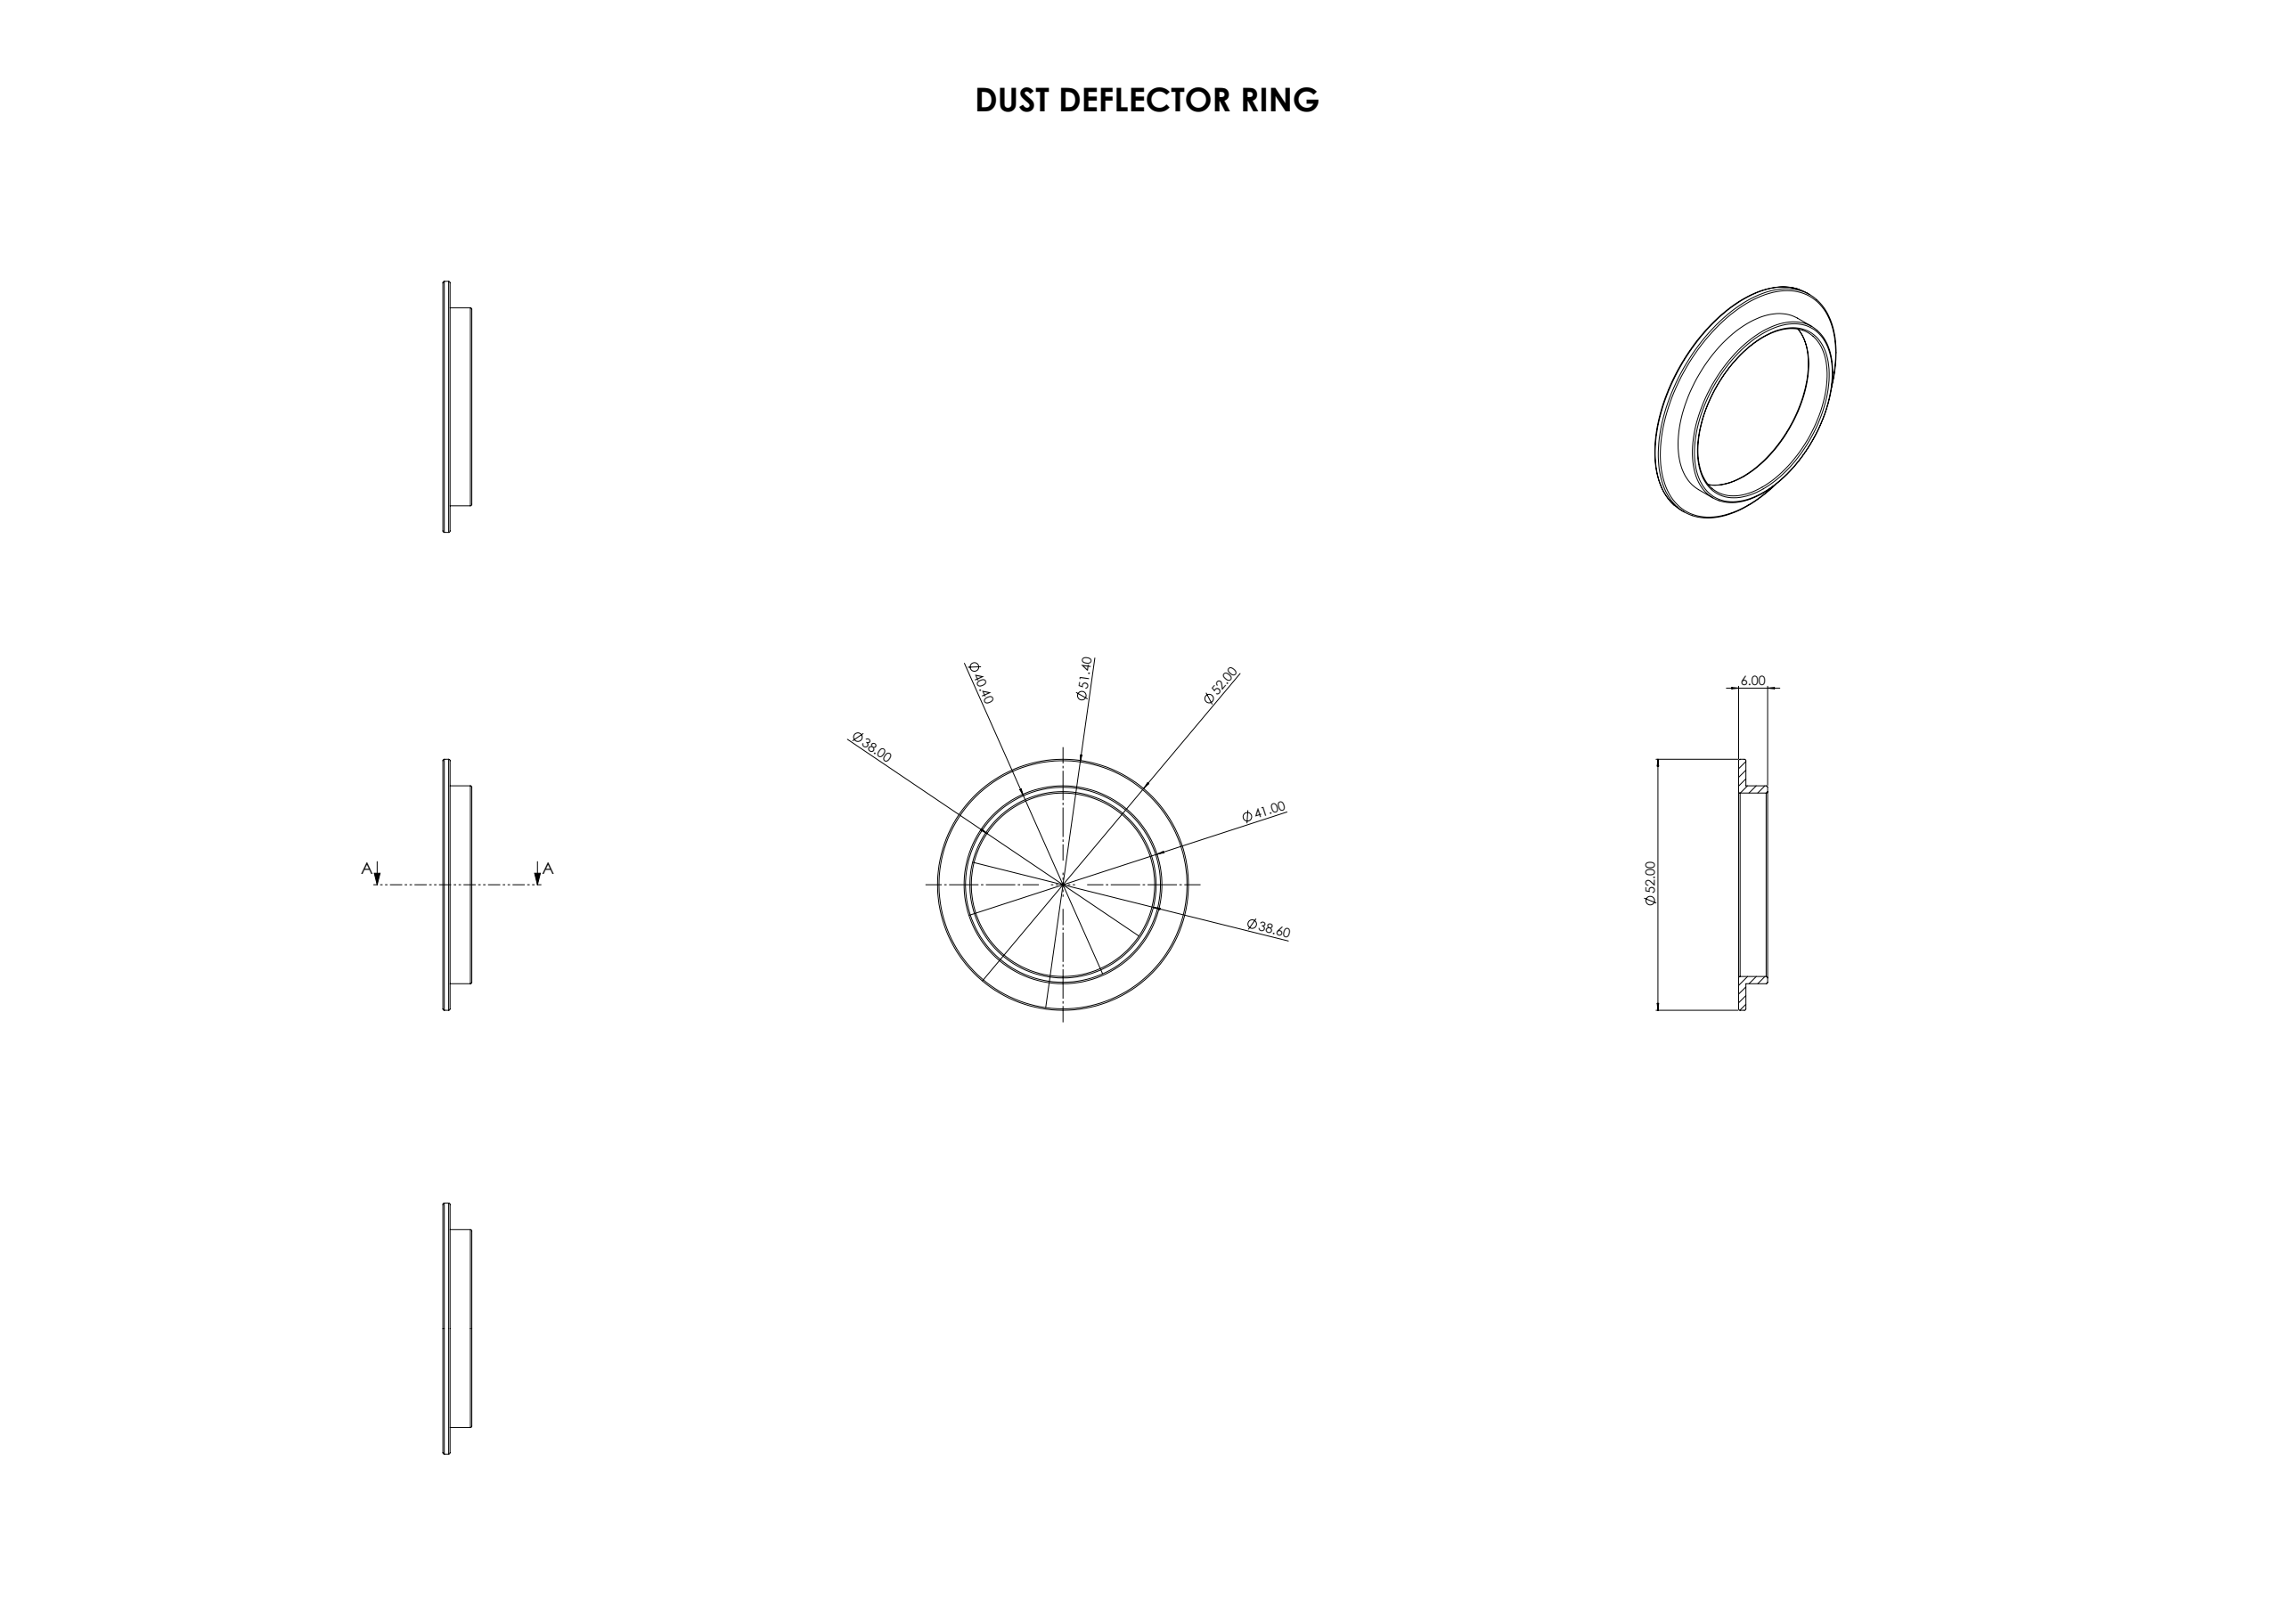
ISO-10303-21;
HEADER;
/* Generated by software containing ST-Developer
 * from STEP Tools, Inc. (www.steptools.com) 
 */

FILE_DESCRIPTION(
/* description */ (''),
/* implementation_level */ '2;1');

FILE_NAME(
/* name */ '16_Dust_Deflector_Ring.step',
/* time_stamp */ '2026-10-11T12:57:03-07:00',
/* author */ (''),
/* organization */ (''),
/* preprocessor_version */ 'ST-DEVELOPER v20.2',
/* originating_system */ 'Autodesk Translation Framework v15.15.0.0',
/* authorisation */ '');

FILE_SCHEMA (('AUTOMOTIVE_DESIGN { 1 0 10303 214 3 1 1 }'));
ENDSEC;

DATA;
#10=MECHANICAL_DESIGN_GEOMETRIC_PRESENTATION_REPRESENTATION('',(#271),#90374);
#237=SHAPE_REPRESENTATION_RELATIONSHIP('SRR','None',#90456,#254);
#254=ADVANCED_BREP_SHAPE_REPRESENTATION('',(#288),#90372);
#271=STYLED_ITEM('',(#90673),#288);
#288=MANIFOLD_SOLID_BREP('Body1',#40360);
#1035=TOROIDAL_SURFACE('',#45228,19.3,0.3);
#1036=TOROIDAL_SURFACE('',#45238,19.3,0.3);
#1037=TOROIDAL_SURFACE('',#45243,20.2,0.3);
#1038=TOROIDAL_SURFACE('',#45249,25.7,0.3);
#1039=TOROIDAL_SURFACE('',#45258,25.7,0.3);
#1113=FACE_BOUND('',#6998,.T.);
#1114=FACE_BOUND('',#7001,.T.);
#1115=FACE_BOUND('',#7007,.T.);
#1821=PLANE('',#45236);
#1822=PLANE('',#45241);
#1823=PLANE('',#45257);
#4525=FACE_OUTER_BOUND('',#6995,.T.);
#4526=FACE_OUTER_BOUND('',#6996,.T.);
#4527=FACE_OUTER_BOUND('',#6997,.T.);
#4528=FACE_OUTER_BOUND('',#6999,.T.);
#4529=FACE_OUTER_BOUND('',#7000,.T.);
#4530=FACE_OUTER_BOUND('',#7002,.T.);
#4531=FACE_OUTER_BOUND('',#7003,.T.);
#4532=FACE_OUTER_BOUND('',#7004,.T.);
#4533=FACE_OUTER_BOUND('',#7005,.T.);
#4534=FACE_OUTER_BOUND('',#7006,.T.);
#4535=FACE_OUTER_BOUND('',#7008,.T.);
#6995=EDGE_LOOP('',(#37155,#37156,#37157,#37158,#37159));
#6996=EDGE_LOOP('',(#37160,#37161,#37162,#37163,#37164,#37165));
#6997=EDGE_LOOP('',(#37166));
#6998=EDGE_LOOP('',(#37167));
#6999=EDGE_LOOP('',(#37168,#37169,#37170,#37171,#37172));
#7000=EDGE_LOOP('',(#37173));
#7001=EDGE_LOOP('',(#37174));
#7002=EDGE_LOOP('',(#37175,#37176,#37177,#37178,#37179));
#7003=EDGE_LOOP('',(#37180,#37181,#37182,#37183,#37184));
#7004=EDGE_LOOP('',(#37185,#37186,#37187,#37188,#37189));
#7005=EDGE_LOOP('',(#37190,#37191,#37192,#37193,#37194,#37195));
#7006=EDGE_LOOP('',(#37196));
#7007=EDGE_LOOP('',(#37197));
#7008=EDGE_LOOP('',(#37198,#37199,#37200,#37201,#37202));
#9399=CIRCLE('',#45229,19.3);
#9400=CIRCLE('',#45230,0.3);
#9401=CIRCLE('',#45231,19.);
#9402=CIRCLE('',#45232,19.);
#9403=CIRCLE('',#45234,19.);
#9404=CIRCLE('',#45235,19.);
#9405=CIRCLE('',#45237,25.7);
#9406=CIRCLE('',#45239,0.3);
#9407=CIRCLE('',#45240,19.3);
#9408=CIRCLE('',#45242,20.2);
#9409=CIRCLE('',#45244,0.3);
#9410=CIRCLE('',#45245,20.5);
#9411=CIRCLE('',#45246,20.5);
#9412=CIRCLE('',#45248,20.5);
#9413=CIRCLE('',#45250,25.7);
#9414=CIRCLE('',#45251,0.3);
#9415=CIRCLE('',#45252,26.);
#9416=CIRCLE('',#45253,26.);
#9417=CIRCLE('',#45255,26.);
#9418=CIRCLE('',#45256,26.);
#9419=CIRCLE('',#45259,0.3);
#12841=LINE('',#90247,#15335);
#12842=LINE('',#90266,#15336);
#12843=LINE('',#90278,#15337);
#15335=VECTOR('',#57151,19.);
#15336=VECTOR('',#57176,20.5);
#15337=VECTOR('',#57191,26.);
#19050=VERTEX_POINT('',#90235);
#19051=VERTEX_POINT('',#90237);
#19052=VERTEX_POINT('',#90239);
#19053=VERTEX_POINT('',#90243);
#19054=VERTEX_POINT('',#90244);
#19055=VERTEX_POINT('',#90249);
#19056=VERTEX_POINT('',#90252);
#19057=VERTEX_POINT('',#90256);
#19058=VERTEX_POINT('',#90259);
#19059=VERTEX_POINT('',#90261);
#19060=VERTEX_POINT('',#90265);
#19061=VERTEX_POINT('',#90269);
#19062=VERTEX_POINT('',#90271);
#19063=VERTEX_POINT('',#90273);
#19064=VERTEX_POINT('',#90277);
#19065=VERTEX_POINT('',#90279);
#25089=EDGE_CURVE('',#19050,#19050,#9399,.T.);
#25090=EDGE_CURVE('',#19050,#19051,#9400,.T.);
#25091=EDGE_CURVE('',#19051,#19052,#9401,.T.);
#25092=EDGE_CURVE('',#19052,#19051,#9402,.T.);
#25093=EDGE_CURVE('',#19053,#19054,#9403,.T.);
#25094=EDGE_CURVE('',#19054,#19053,#9404,.T.);
#25095=EDGE_CURVE('',#19054,#19052,#12841,.T.);
#25096=EDGE_CURVE('',#19055,#19055,#9405,.T.);
#25097=EDGE_CURVE('',#19053,#19056,#9406,.T.);
#25098=EDGE_CURVE('',#19056,#19056,#9407,.T.);
#25099=EDGE_CURVE('',#19057,#19057,#9408,.T.);
#25100=EDGE_CURVE('',#19057,#19058,#9409,.T.);
#25101=EDGE_CURVE('',#19058,#19059,#9410,.T.);
#25102=EDGE_CURVE('',#19059,#19058,#9411,.T.);
#25103=EDGE_CURVE('',#19059,#19060,#12842,.T.);
#25104=EDGE_CURVE('',#19060,#19060,#9412,.T.);
#25105=EDGE_CURVE('',#19061,#19061,#9413,.T.);
#25106=EDGE_CURVE('',#19061,#19062,#9414,.T.);
#25107=EDGE_CURVE('',#19062,#19063,#9415,.T.);
#25108=EDGE_CURVE('',#19063,#19062,#9416,.T.);
#25109=EDGE_CURVE('',#19063,#19064,#12843,.T.);
#25110=EDGE_CURVE('',#19065,#19064,#9417,.T.);
#25111=EDGE_CURVE('',#19064,#19065,#9418,.T.);
#25112=EDGE_CURVE('',#19065,#19055,#9419,.T.);
#37155=ORIENTED_EDGE('',*,*,#25089,.T.);
#37156=ORIENTED_EDGE('',*,*,#25090,.T.);
#37157=ORIENTED_EDGE('',*,*,#25091,.T.);
#37158=ORIENTED_EDGE('',*,*,#25092,.T.);
#37159=ORIENTED_EDGE('',*,*,#25090,.F.);
#37160=ORIENTED_EDGE('',*,*,#25093,.F.);
#37161=ORIENTED_EDGE('',*,*,#25094,.F.);
#37162=ORIENTED_EDGE('',*,*,#25095,.T.);
#37163=ORIENTED_EDGE('',*,*,#25091,.F.);
#37164=ORIENTED_EDGE('',*,*,#25092,.F.);
#37165=ORIENTED_EDGE('',*,*,#25095,.F.);
#37166=ORIENTED_EDGE('',*,*,#25096,.F.);
#37167=ORIENTED_EDGE('',*,*,#25089,.F.);
#37168=ORIENTED_EDGE('',*,*,#25093,.T.);
#37169=ORIENTED_EDGE('',*,*,#25094,.T.);
#37170=ORIENTED_EDGE('',*,*,#25097,.T.);
#37171=ORIENTED_EDGE('',*,*,#25098,.T.);
#37172=ORIENTED_EDGE('',*,*,#25097,.F.);
#37173=ORIENTED_EDGE('',*,*,#25099,.F.);
#37174=ORIENTED_EDGE('',*,*,#25098,.F.);
#37175=ORIENTED_EDGE('',*,*,#25099,.T.);
#37176=ORIENTED_EDGE('',*,*,#25100,.T.);
#37177=ORIENTED_EDGE('',*,*,#25101,.T.);
#37178=ORIENTED_EDGE('',*,*,#25102,.T.);
#37179=ORIENTED_EDGE('',*,*,#25100,.F.);
#37180=ORIENTED_EDGE('',*,*,#25102,.F.);
#37181=ORIENTED_EDGE('',*,*,#25103,.T.);
#37182=ORIENTED_EDGE('',*,*,#25104,.T.);
#37183=ORIENTED_EDGE('',*,*,#25103,.F.);
#37184=ORIENTED_EDGE('',*,*,#25101,.F.);
#37185=ORIENTED_EDGE('',*,*,#25105,.T.);
#37186=ORIENTED_EDGE('',*,*,#25106,.T.);
#37187=ORIENTED_EDGE('',*,*,#25107,.T.);
#37188=ORIENTED_EDGE('',*,*,#25108,.T.);
#37189=ORIENTED_EDGE('',*,*,#25106,.F.);
#37190=ORIENTED_EDGE('',*,*,#25108,.F.);
#37191=ORIENTED_EDGE('',*,*,#25109,.T.);
#37192=ORIENTED_EDGE('',*,*,#25110,.F.);
#37193=ORIENTED_EDGE('',*,*,#25111,.F.);
#37194=ORIENTED_EDGE('',*,*,#25109,.F.);
#37195=ORIENTED_EDGE('',*,*,#25107,.F.);
#37196=ORIENTED_EDGE('',*,*,#25105,.F.);
#37197=ORIENTED_EDGE('',*,*,#25104,.F.);
#37198=ORIENTED_EDGE('',*,*,#25110,.T.);
#37199=ORIENTED_EDGE('',*,*,#25111,.T.);
#37200=ORIENTED_EDGE('',*,*,#25112,.T.);
#37201=ORIENTED_EDGE('',*,*,#25096,.T.);
#37202=ORIENTED_EDGE('',*,*,#25112,.F.);
#37943=CYLINDRICAL_SURFACE('',#45233,19.);
#37944=CYLINDRICAL_SURFACE('',#45247,20.5);
#37945=CYLINDRICAL_SURFACE('',#45254,26.);
#40328=ADVANCED_FACE('',(#4525),#1035,.T.);
#40329=ADVANCED_FACE('',(#4526),#37943,.F.);
#40330=ADVANCED_FACE('',(#4527,#1113),#1821,.T.);
#40331=ADVANCED_FACE('',(#4528),#1036,.T.);
#40332=ADVANCED_FACE('',(#4529,#1114),#1822,.T.);
#40333=ADVANCED_FACE('',(#4530),#1037,.T.);
#40334=ADVANCED_FACE('',(#4531),#37944,.T.);
#40335=ADVANCED_FACE('',(#4532),#1038,.T.);
#40336=ADVANCED_FACE('',(#4533),#37945,.T.);
#40337=ADVANCED_FACE('',(#4534,#1115),#1823,.T.);
#40338=ADVANCED_FACE('',(#4535),#1039,.T.);
#40360=CLOSED_SHELL('',(#40328,#40329,#40330,#40331,#40332,#40333,#40334,
#40335,#40336,#40337,#40338));
#45227=AXIS2_PLACEMENT_3D('',#90233,#57133,#57134);
#45228=AXIS2_PLACEMENT_3D('',#90234,#57135,#57136);
#45229=AXIS2_PLACEMENT_3D('',#90236,#57137,#57138);
#45230=AXIS2_PLACEMENT_3D('',#90238,#57139,#57140);
#45231=AXIS2_PLACEMENT_3D('',#90240,#57141,#57142);
#45232=AXIS2_PLACEMENT_3D('',#90241,#57143,#57144);
#45233=AXIS2_PLACEMENT_3D('',#90242,#57145,#57146);
#45234=AXIS2_PLACEMENT_3D('',#90245,#57147,#57148);
#45235=AXIS2_PLACEMENT_3D('',#90246,#57149,#57150);
#45236=AXIS2_PLACEMENT_3D('',#90248,#57152,#57153);
#45237=AXIS2_PLACEMENT_3D('',#90250,#57154,#57155);
#45238=AXIS2_PLACEMENT_3D('',#90251,#57156,#57157);
#45239=AXIS2_PLACEMENT_3D('',#90253,#57158,#57159);
#45240=AXIS2_PLACEMENT_3D('',#90254,#57160,#57161);
#45241=AXIS2_PLACEMENT_3D('',#90255,#57162,#57163);
#45242=AXIS2_PLACEMENT_3D('',#90257,#57164,#57165);
#45243=AXIS2_PLACEMENT_3D('',#90258,#57166,#57167);
#45244=AXIS2_PLACEMENT_3D('',#90260,#57168,#57169);
#45245=AXIS2_PLACEMENT_3D('',#90262,#57170,#57171);
#45246=AXIS2_PLACEMENT_3D('',#90263,#57172,#57173);
#45247=AXIS2_PLACEMENT_3D('',#90264,#57174,#57175);
#45248=AXIS2_PLACEMENT_3D('',#90267,#57177,#57178);
#45249=AXIS2_PLACEMENT_3D('',#90268,#57179,#57180);
#45250=AXIS2_PLACEMENT_3D('',#90270,#57181,#57182);
#45251=AXIS2_PLACEMENT_3D('',#90272,#57183,#57184);
#45252=AXIS2_PLACEMENT_3D('',#90274,#57185,#57186);
#45253=AXIS2_PLACEMENT_3D('',#90275,#57187,#57188);
#45254=AXIS2_PLACEMENT_3D('',#90276,#57189,#57190);
#45255=AXIS2_PLACEMENT_3D('',#90280,#57192,#57193);
#45256=AXIS2_PLACEMENT_3D('',#90281,#57194,#57195);
#45257=AXIS2_PLACEMENT_3D('',#90282,#57196,#57197);
#45258=AXIS2_PLACEMENT_3D('',#90283,#57198,#57199);
#45259=AXIS2_PLACEMENT_3D('',#90284,#57200,#57201);
#57133=DIRECTION('axis',(0.,0.,1.));
#57134=DIRECTION('refdir',(1.,0.,0.));
#57135=DIRECTION('center_axis',(1.,0.,0.));
#57136=DIRECTION('ref_axis',(0.,0.,-1.));
#57137=DIRECTION('center_axis',(-1.,0.,0.));
#57138=DIRECTION('ref_axis',(0.,-1.,1.83697019872103E-16));
#57139=DIRECTION('center_axis',(0.,-1.,-1.22464679914735E-16));
#57140=DIRECTION('ref_axis',(0.,-1.22464679914735E-16,1.));
#57141=DIRECTION('center_axis',(1.,0.,0.));
#57142=DIRECTION('ref_axis',(0.,-1.,1.83697019872103E-16));
#57143=DIRECTION('center_axis',(1.,0.,0.));
#57144=DIRECTION('ref_axis',(0.,-1.,1.83697019872103E-16));
#57145=DIRECTION('center_axis',(1.,0.,0.));
#57146=DIRECTION('ref_axis',(0.,1.,0.));
#57147=DIRECTION('center_axis',(-1.,0.,0.));
#57148=DIRECTION('ref_axis',(0.,-1.,1.83697019872103E-16));
#57149=DIRECTION('center_axis',(-1.,0.,0.));
#57150=DIRECTION('ref_axis',(0.,-1.,1.83697019872103E-16));
#57151=DIRECTION('',(-1.,0.,0.));
#57152=DIRECTION('center_axis',(-1.,0.,0.));
#57153=DIRECTION('ref_axis',(0.,0.,1.));
#57154=DIRECTION('center_axis',(1.,0.,0.));
#57155=DIRECTION('ref_axis',(0.,-1.,1.83697019872103E-16));
#57156=DIRECTION('center_axis',(1.,0.,0.));
#57157=DIRECTION('ref_axis',(0.,0.,-1.));
#57158=DIRECTION('center_axis',(0.,-1.,-1.22464679914735E-16));
#57159=DIRECTION('ref_axis',(0.,-1.22464679914735E-16,1.));
#57160=DIRECTION('center_axis',(1.,0.,0.));
#57161=DIRECTION('ref_axis',(0.,-1.,1.83697019872103E-16));
#57162=DIRECTION('center_axis',(1.,0.,0.));
#57163=DIRECTION('ref_axis',(0.,0.,-1.));
#57164=DIRECTION('center_axis',(-1.,0.,0.));
#57165=DIRECTION('ref_axis',(0.,-1.,1.83697019872103E-16));
#57166=DIRECTION('center_axis',(1.,0.,0.));
#57167=DIRECTION('ref_axis',(0.,0.,-1.));
#57168=DIRECTION('center_axis',(0.,-1.,-1.22464679914735E-16));
#57169=DIRECTION('ref_axis',(0.,-1.22464679914735E-16,1.));
#57170=DIRECTION('center_axis',(1.,0.,0.));
#57171=DIRECTION('ref_axis',(0.,-1.,1.83697019872103E-16));
#57172=DIRECTION('center_axis',(1.,0.,0.));
#57173=DIRECTION('ref_axis',(0.,-1.,1.83697019872103E-16));
#57174=DIRECTION('center_axis',(1.,0.,0.));
#57175=DIRECTION('ref_axis',(0.,1.,0.));
#57176=DIRECTION('',(-1.,0.,0.));
#57177=DIRECTION('center_axis',(1.,0.,0.));
#57178=DIRECTION('ref_axis',(0.,0.,-1.));
#57179=DIRECTION('center_axis',(1.,0.,0.));
#57180=DIRECTION('ref_axis',(0.,0.,-1.));
#57181=DIRECTION('center_axis',(-1.,0.,0.));
#57182=DIRECTION('ref_axis',(0.,-1.,1.83697019872103E-16));
#57183=DIRECTION('center_axis',(0.,-1.,-1.22464679914735E-16));
#57184=DIRECTION('ref_axis',(0.,-1.22464679914735E-16,1.));
#57185=DIRECTION('center_axis',(1.,0.,0.));
#57186=DIRECTION('ref_axis',(0.,-1.,1.83697019872103E-16));
#57187=DIRECTION('center_axis',(1.,0.,0.));
#57188=DIRECTION('ref_axis',(0.,-1.,1.83697019872103E-16));
#57189=DIRECTION('center_axis',(1.,0.,0.));
#57190=DIRECTION('ref_axis',(0.,1.,0.));
#57191=DIRECTION('',(-1.,0.,0.));
#57192=DIRECTION('center_axis',(-1.,0.,0.));
#57193=DIRECTION('ref_axis',(0.,-1.,1.83697019872103E-16));
#57194=DIRECTION('center_axis',(-1.,0.,0.));
#57195=DIRECTION('ref_axis',(0.,-1.,1.83697019872103E-16));
#57196=DIRECTION('center_axis',(1.,0.,0.));
#57197=DIRECTION('ref_axis',(0.,0.,-1.));
#57198=DIRECTION('center_axis',(1.,0.,0.));
#57199=DIRECTION('ref_axis',(0.,0.,-1.));
#57200=DIRECTION('center_axis',(0.,-1.,-1.22464679914735E-16));
#57201=DIRECTION('ref_axis',(0.,-1.22464679914735E-16,1.));
#90233=CARTESIAN_POINT('',(0.,0.,0.));
#90234=CARTESIAN_POINT('Origin',(588.3,0.,0.));
#90235=CARTESIAN_POINT('',(588.,-2.36356832235439E-15,19.3));
#90236=CARTESIAN_POINT('Origin',(588.,0.,0.));
#90237=CARTESIAN_POINT('',(588.3,-2.32682891837997E-15,19.));
#90238=CARTESIAN_POINT('Origin',(588.3,-2.36356832235439E-15,19.3));
#90239=CARTESIAN_POINT('',(588.3,-19.,-2.32682891837997E-15));
#90240=CARTESIAN_POINT('Origin',(588.3,0.,0.));
#90241=CARTESIAN_POINT('Origin',(588.3,0.,0.));
#90242=CARTESIAN_POINT('Origin',(591.,0.,0.));
#90243=CARTESIAN_POINT('',(593.7,-2.32682891837997E-15,19.));
#90244=CARTESIAN_POINT('',(593.7,-19.,-2.32682891837997E-15));
#90245=CARTESIAN_POINT('Origin',(593.7,0.,0.));
#90246=CARTESIAN_POINT('Origin',(593.7,0.,0.));
#90247=CARTESIAN_POINT('',(591.,-19.,-2.32682891837997E-15));
#90248=CARTESIAN_POINT('Origin',(588.,26.,0.));
#90249=CARTESIAN_POINT('',(588.,-3.1473422738087E-15,25.7));
#90250=CARTESIAN_POINT('Origin',(588.,0.,0.));
#90251=CARTESIAN_POINT('Origin',(593.7,0.,0.));
#90252=CARTESIAN_POINT('',(594.,-2.36356832235439E-15,19.3));
#90253=CARTESIAN_POINT('Origin',(593.7,-2.36356832235439E-15,19.3));
#90254=CARTESIAN_POINT('Origin',(594.,0.,0.));
#90255=CARTESIAN_POINT('Origin',(594.,19.,0.));
#90256=CARTESIAN_POINT('',(594.,-2.47378653427765E-15,20.2));
#90257=CARTESIAN_POINT('Origin',(594.,0.,0.));
#90258=CARTESIAN_POINT('Origin',(593.7,0.,0.));
#90259=CARTESIAN_POINT('',(593.7,-2.51052593825207E-15,20.5));
#90260=CARTESIAN_POINT('Origin',(593.7,-2.47378653427765E-15,20.2));
#90261=CARTESIAN_POINT('',(593.7,-20.5,-2.51052593825207E-15));
#90262=CARTESIAN_POINT('Origin',(593.7,0.,0.));
#90263=CARTESIAN_POINT('Origin',(593.7,0.,0.));
#90264=CARTESIAN_POINT('Origin',(591.75,0.,0.));
#90265=CARTESIAN_POINT('',(589.5,-20.5,-2.51052593825207E-15));
#90266=CARTESIAN_POINT('',(591.75,-20.5,-2.51052593825207E-15));
#90267=CARTESIAN_POINT('Origin',(589.5,0.,0.));
#90268=CARTESIAN_POINT('Origin',(589.2,0.,0.));
#90269=CARTESIAN_POINT('',(589.5,-3.1473422738087E-15,25.7));
#90270=CARTESIAN_POINT('Origin',(589.5,0.,0.));
#90271=CARTESIAN_POINT('',(589.2,-3.18408167778312E-15,26.));
#90272=CARTESIAN_POINT('Origin',(589.2,-3.1473422738087E-15,25.7));
#90273=CARTESIAN_POINT('',(589.2,-26.,-3.18408167778312E-15));
#90274=CARTESIAN_POINT('Origin',(589.2,0.,0.));
#90275=CARTESIAN_POINT('Origin',(589.2,0.,0.));
#90276=CARTESIAN_POINT('Origin',(588.75,0.,0.));
#90277=CARTESIAN_POINT('',(588.3,-26.,-3.18408167778312E-15));
#90278=CARTESIAN_POINT('',(588.75,-26.,-3.18408167778312E-15));
#90279=CARTESIAN_POINT('',(588.3,-3.18408167778312E-15,26.));
#90280=CARTESIAN_POINT('Origin',(588.3,0.,0.));
#90281=CARTESIAN_POINT('Origin',(588.3,0.,0.));
#90282=CARTESIAN_POINT('Origin',(589.5,20.5,0.));
#90283=CARTESIAN_POINT('Origin',(588.3,0.,0.));
#90284=CARTESIAN_POINT('Origin',(588.3,-3.1473422738087E-15,25.7));
#90353=UNCERTAINTY_MEASURE_WITH_UNIT(LENGTH_MEASURE(0.01),#90375,
'DISTANCE_ACCURACY_VALUE',
'Maximum model space distance between geometric entities at asserted c
onnectivities');
#90355=UNCERTAINTY_MEASURE_WITH_UNIT(LENGTH_MEASURE(0.01),#90375,
'DISTANCE_ACCURACY_VALUE',
'Maximum model space distance between geometric entities at asserted c
onnectivities');
#90372=(
GEOMETRIC_REPRESENTATION_CONTEXT(3)
GLOBAL_UNCERTAINTY_ASSIGNED_CONTEXT((#90353))
GLOBAL_UNIT_ASSIGNED_CONTEXT((#90375,#90377,#90378))
REPRESENTATION_CONTEXT('','3D')
);
#90374=(
GEOMETRIC_REPRESENTATION_CONTEXT(3)
GLOBAL_UNCERTAINTY_ASSIGNED_CONTEXT((#90355))
GLOBAL_UNIT_ASSIGNED_CONTEXT((#90375,#90377,#90378))
REPRESENTATION_CONTEXT('','3D')
);
#90375=(
LENGTH_UNIT()
NAMED_UNIT(*)
SI_UNIT(.MILLI.,.METRE.)
);
#90377=(
NAMED_UNIT(*)
PLANE_ANGLE_UNIT()
SI_UNIT($,.RADIAN.)
);
#90378=(
NAMED_UNIT(*)
SI_UNIT($,.STERADIAN.)
SOLID_ANGLE_UNIT()
);
#90395=SHAPE_DEFINITION_REPRESENTATION(#90413,#90456);
#90413=PRODUCT_DEFINITION_SHAPE('',$,#90475);
#90456=SHAPE_REPRESENTATION('',(#45227),#90372);
#90458=PRODUCT_DEFINITION_CONTEXT('part definition',#90514,'design');
#90475=PRODUCT_DEFINITION('2026-10-11-12-53-16-239',
'16_Dust_Deflector_Ring',#90493,#90458);
#90493=PRODUCT_DEFINITION_FORMATION('',$,#90532);
#90514=APPLICATION_CONTEXT(
'Core Data for Automotive Mechanical Design Process');
#90515=PRODUCT_CONTEXT('part definition',#90514,'mechanical');
#90532=PRODUCT('2026-10-11-12-53-16-239','16_Dust_Deflector_Ring',$,(#90515));
#90667=COLOUR_RGB('Light Blue',0.38,0.62,0.78);
#90668=FILL_AREA_STYLE_COLOUR('',#90667);
#90669=FILL_AREA_STYLE('',(#90668));
#90670=SURFACE_STYLE_FILL_AREA(#90669);
#90671=SURFACE_SIDE_STYLE('',(#90670));
#90672=SURFACE_STYLE_USAGE(.BOTH.,#90671);
#90673=PRESENTATION_STYLE_ASSIGNMENT((#90672));
ENDSEC;
END-ISO-10303-21;
